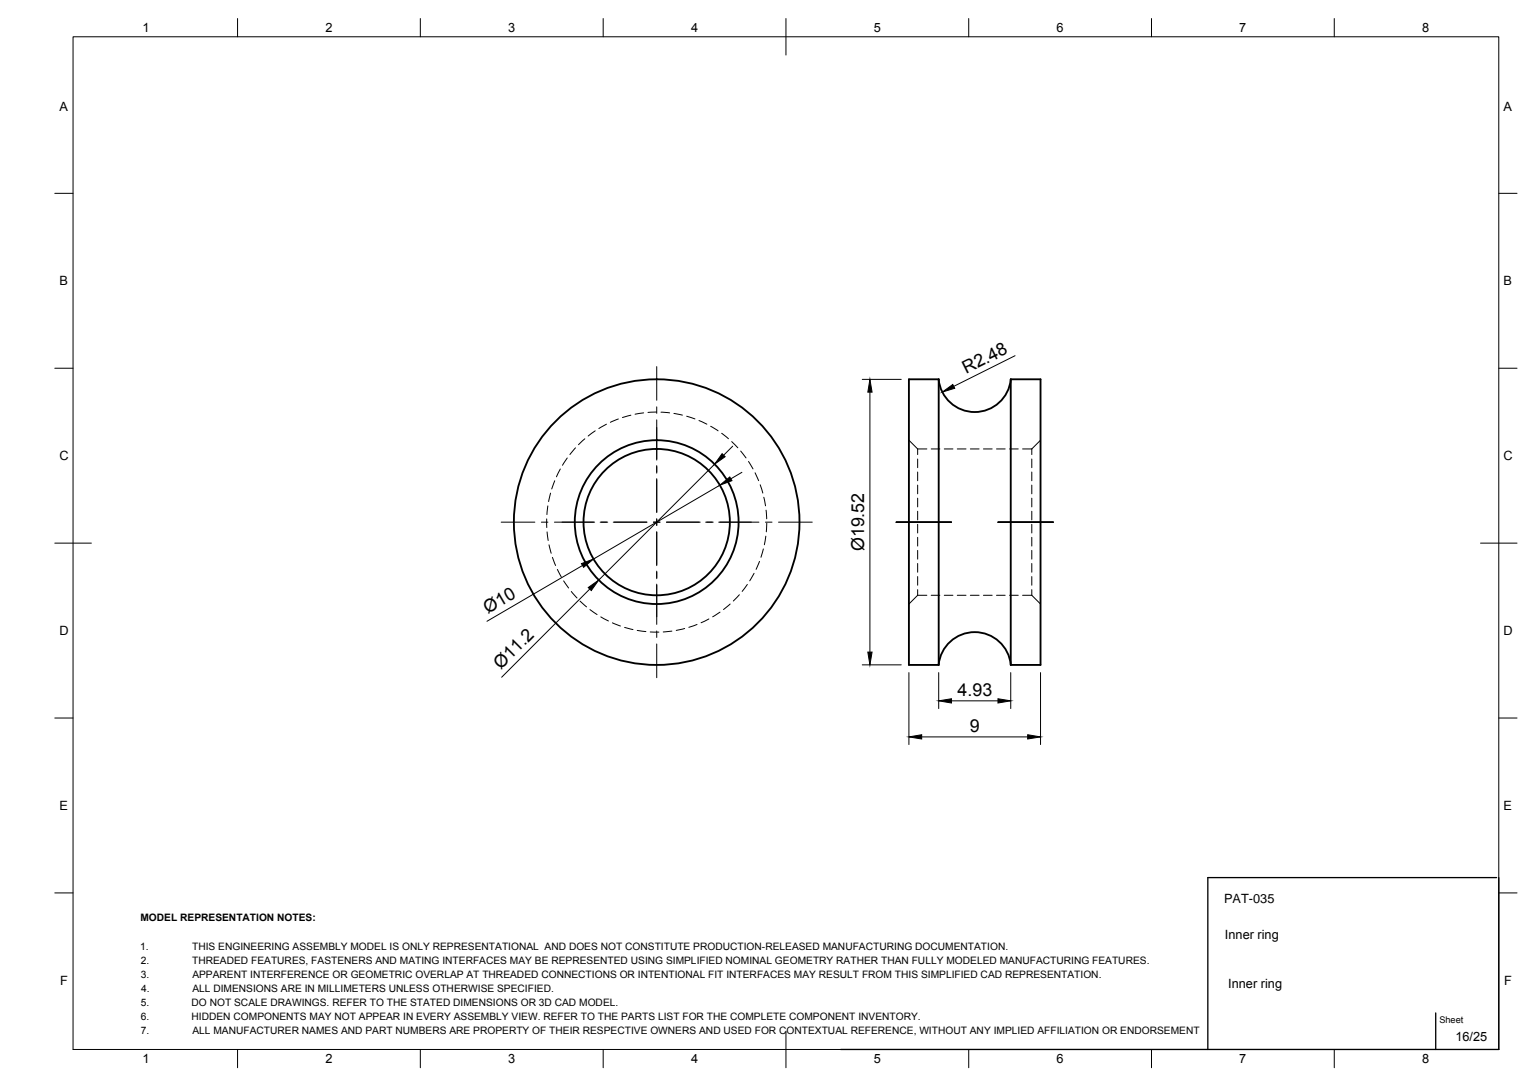
ISO-10303-21;
HEADER;
/* Generated by software containing ST-Developer
 * from STEP Tools, Inc. (www.steptools.com) 
 */

FILE_DESCRIPTION(
/* description */ ('Five-roller gravity conveyor'),
/* implementation_level */ '2;1');

FILE_NAME(
/* name */ 'Inner ring.step',
/* time_stamp */ '2026-10-29T15:36:43-07:00',
/* author */ (''),
/* organization */ (''),
/* preprocessor_version */ 'ST-DEVELOPER v20.2',
/* originating_system */ 'Autodesk Translation Framework v15.17.0.0',
/* authorisation */ '');

FILE_SCHEMA (('AUTOMOTIVE_DESIGN { 1 0 10303 214 3 1 1 }'));
ENDSEC;

DATA;
#10=MECHANICAL_DESIGN_GEOMETRIC_PRESENTATION_REPRESENTATION('',(#318),#7806);
#257=TOROIDAL_SURFACE('',#4620,1.,0.247676);
#264=CONICAL_SURFACE('',#4631,0.53,0.785398163397448);
#265=CONICAL_SURFACE('',#4638,0.53,0.785398163397448);
#282=SHAPE_REPRESENTATION_RELATIONSHIP('SRR','None',#7920,#300);
#300=ADVANCED_BREP_SHAPE_REPRESENTATION('',(#343),#7793);
#318=STYLED_ITEM('',(#8091),#343);
#343=MANIFOLD_SOLID_BREP('Body1',#4206);
#382=FACE_BOUND('',#1039,.T.);
#383=FACE_BOUND('',#1042,.T.);
#472=CIRCLE('',#4621,0.976185);
#473=CIRCLE('',#4622,0.976185);
#474=CIRCLE('',#4623,0.247676);
#475=CIRCLE('',#4624,0.976185);
#476=CIRCLE('',#4625,0.976185);
#477=CIRCLE('',#4627,0.976185);
#478=CIRCLE('',#4629,0.5);
#479=CIRCLE('',#4630,0.5);
#480=CIRCLE('',#4632,0.56);
#481=CIRCLE('',#4635,0.976185);
#482=CIRCLE('',#4637,0.56);
#617=CYLINDRICAL_SURFACE('',#4626,0.976185);
#618=CYLINDRICAL_SURFACE('',#4628,0.5);
#619=CYLINDRICAL_SURFACE('',#4634,0.976185);
#782=FACE_OUTER_BOUND('',#1034,.T.);
#783=FACE_OUTER_BOUND('',#1035,.T.);
#784=FACE_OUTER_BOUND('',#1036,.T.);
#785=FACE_OUTER_BOUND('',#1037,.T.);
#786=FACE_OUTER_BOUND('',#1038,.T.);
#787=FACE_OUTER_BOUND('',#1040,.T.);
#788=FACE_OUTER_BOUND('',#1041,.T.);
#789=FACE_OUTER_BOUND('',#1043,.T.);
#1034=EDGE_LOOP('',(#3420,#3421,#3422,#3423,#3424,#3425));
#1035=EDGE_LOOP('',(#3426,#3427,#3428,#3429,#3430));
#1036=EDGE_LOOP('',(#3431,#3432,#3433,#3434));
#1037=EDGE_LOOP('',(#3435,#3436,#3437,#3438));
#1038=EDGE_LOOP('',(#3439));
#1039=EDGE_LOOP('',(#3440));
#1040=EDGE_LOOP('',(#3441,#3442,#3443,#3444,#3445));
#1041=EDGE_LOOP('',(#3446));
#1042=EDGE_LOOP('',(#3447));
#1043=EDGE_LOOP('',(#3448,#3449,#3450,#3451));
#1455=LINE('',#6923,#1796);
#1456=LINE('',#6929,#1797);
#1457=LINE('',#6933,#1798);
#1458=LINE('',#6939,#1799);
#1459=LINE('',#6944,#1800);
#1796=VECTOR('',#5591,0.976185);
#1797=VECTOR('',#5598,0.5);
#1798=VECTOR('',#5603,0.53);
#1799=VECTOR('',#5612,0.976185);
#1800=VECTOR('',#5619,0.53);
#2078=VERTEX_POINT('',#6912);
#2079=VERTEX_POINT('',#6913);
#2080=VERTEX_POINT('',#6916);
#2081=VERTEX_POINT('',#6918);
#2082=VERTEX_POINT('',#6922);
#2083=VERTEX_POINT('',#6926);
#2084=VERTEX_POINT('',#6928);
#2085=VERTEX_POINT('',#6932);
#2086=VERTEX_POINT('',#6937);
#2087=VERTEX_POINT('',#6941);
#2553=EDGE_CURVE('',#2078,#2079,#472,.T.);
#2554=EDGE_CURVE('',#2079,#2078,#473,.T.);
#2555=EDGE_CURVE('',#2079,#2080,#474,.T.);
#2556=EDGE_CURVE('',#2081,#2080,#475,.T.);
#2557=EDGE_CURVE('',#2080,#2081,#476,.T.);
#2558=EDGE_CURVE('',#2081,#2082,#1455,.T.);
#2559=EDGE_CURVE('',#2082,#2082,#477,.T.);
#2560=EDGE_CURVE('',#2083,#2083,#478,.T.);
#2561=EDGE_CURVE('',#2083,#2084,#1456,.T.);
#2562=EDGE_CURVE('',#2084,#2084,#479,.T.);
#2563=EDGE_CURVE('',#2084,#2085,#1457,.T.);
#2564=EDGE_CURVE('',#2085,#2085,#480,.T.);
#2565=EDGE_CURVE('',#2086,#2086,#481,.T.);
#2566=EDGE_CURVE('',#2086,#2078,#1458,.T.);
#2567=EDGE_CURVE('',#2087,#2087,#482,.T.);
#2568=EDGE_CURVE('',#2087,#2083,#1459,.T.);
#3420=ORIENTED_EDGE('',*,*,#2553,.F.);
#3421=ORIENTED_EDGE('',*,*,#2554,.F.);
#3422=ORIENTED_EDGE('',*,*,#2555,.T.);
#3423=ORIENTED_EDGE('',*,*,#2556,.F.);
#3424=ORIENTED_EDGE('',*,*,#2557,.F.);
#3425=ORIENTED_EDGE('',*,*,#2555,.F.);
#3426=ORIENTED_EDGE('',*,*,#2556,.T.);
#3427=ORIENTED_EDGE('',*,*,#2557,.T.);
#3428=ORIENTED_EDGE('',*,*,#2558,.T.);
#3429=ORIENTED_EDGE('',*,*,#2559,.T.);
#3430=ORIENTED_EDGE('',*,*,#2558,.F.);
#3431=ORIENTED_EDGE('',*,*,#2560,.T.);
#3432=ORIENTED_EDGE('',*,*,#2561,.T.);
#3433=ORIENTED_EDGE('',*,*,#2562,.F.);
#3434=ORIENTED_EDGE('',*,*,#2561,.F.);
#3435=ORIENTED_EDGE('',*,*,#2562,.T.);
#3436=ORIENTED_EDGE('',*,*,#2563,.T.);
#3437=ORIENTED_EDGE('',*,*,#2564,.F.);
#3438=ORIENTED_EDGE('',*,*,#2563,.F.);
#3439=ORIENTED_EDGE('',*,*,#2559,.F.);
#3440=ORIENTED_EDGE('',*,*,#2564,.T.);
#3441=ORIENTED_EDGE('',*,*,#2565,.F.);
#3442=ORIENTED_EDGE('',*,*,#2566,.T.);
#3443=ORIENTED_EDGE('',*,*,#2553,.T.);
#3444=ORIENTED_EDGE('',*,*,#2554,.T.);
#3445=ORIENTED_EDGE('',*,*,#2566,.F.);
#3446=ORIENTED_EDGE('',*,*,#2565,.T.);
#3447=ORIENTED_EDGE('',*,*,#2567,.F.);
#3448=ORIENTED_EDGE('',*,*,#2567,.T.);
#3449=ORIENTED_EDGE('',*,*,#2568,.T.);
#3450=ORIENTED_EDGE('',*,*,#2560,.F.);
#3451=ORIENTED_EDGE('',*,*,#2568,.F.);
#3926=PLANE('',#4633);
#3927=PLANE('',#4636);
#4097=ADVANCED_FACE('',(#782),#257,.F.);
#4098=ADVANCED_FACE('',(#783),#617,.T.);
#4099=ADVANCED_FACE('',(#784),#618,.F.);
#4100=ADVANCED_FACE('',(#785),#264,.F.);
#4101=ADVANCED_FACE('',(#786,#382),#3926,.T.);
#4102=ADVANCED_FACE('',(#787),#619,.T.);
#4103=ADVANCED_FACE('',(#788,#383),#3927,.T.);
#4104=ADVANCED_FACE('',(#789),#265,.F.);
#4206=CLOSED_SHELL('',(#4097,#4098,#4099,#4100,#4101,#4102,#4103,#4104));
#4619=AXIS2_PLACEMENT_3D('',#6910,#5575,#5576);
#4620=AXIS2_PLACEMENT_3D('',#6911,#5577,#5578);
#4621=AXIS2_PLACEMENT_3D('',#6914,#5579,#5580);
#4622=AXIS2_PLACEMENT_3D('',#6915,#5581,#5582);
#4623=AXIS2_PLACEMENT_3D('',#6917,#5583,#5584);
#4624=AXIS2_PLACEMENT_3D('',#6919,#5585,#5586);
#4625=AXIS2_PLACEMENT_3D('',#6920,#5587,#5588);
#4626=AXIS2_PLACEMENT_3D('',#6921,#5589,#5590);
#4627=AXIS2_PLACEMENT_3D('',#6924,#5592,#5593);
#4628=AXIS2_PLACEMENT_3D('',#6925,#5594,#5595);
#4629=AXIS2_PLACEMENT_3D('',#6927,#5596,#5597);
#4630=AXIS2_PLACEMENT_3D('',#6930,#5599,#5600);
#4631=AXIS2_PLACEMENT_3D('',#6931,#5601,#5602);
#4632=AXIS2_PLACEMENT_3D('',#6934,#5604,#5605);
#4633=AXIS2_PLACEMENT_3D('',#6935,#5606,#5607);
#4634=AXIS2_PLACEMENT_3D('',#6936,#5608,#5609);
#4635=AXIS2_PLACEMENT_3D('',#6938,#5610,#5611);
#4636=AXIS2_PLACEMENT_3D('',#6940,#5613,#5614);
#4637=AXIS2_PLACEMENT_3D('',#6942,#5615,#5616);
#4638=AXIS2_PLACEMENT_3D('',#6943,#5617,#5618);
#5575=DIRECTION('axis',(0.,0.,1.));
#5576=DIRECTION('refdir',(1.,0.,0.));
#5577=DIRECTION('center_axis',(0.,-1.,0.));
#5578=DIRECTION('ref_axis',(0.,0.,-1.));
#5579=DIRECTION('center_axis',(0.,-1.,0.));
#5580=DIRECTION('ref_axis',(1.,0.,0.));
#5581=DIRECTION('center_axis',(0.,-1.,0.));
#5582=DIRECTION('ref_axis',(1.,0.,0.));
#5583=DIRECTION('center_axis',(1.,0.,1.22464679914735E-16));
#5584=DIRECTION('ref_axis',(-1.22464679914735E-16,0.,1.));
#5585=DIRECTION('center_axis',(0.,1.,0.));
#5586=DIRECTION('ref_axis',(1.,0.,0.));
#5587=DIRECTION('center_axis',(0.,1.,0.));
#5588=DIRECTION('ref_axis',(1.,0.,0.));
#5589=DIRECTION('center_axis',(0.,-1.,0.));
#5590=DIRECTION('ref_axis',(1.,0.,0.));
#5591=DIRECTION('',(0.,1.,0.));
#5592=DIRECTION('center_axis',(0.,-1.,0.));
#5593=DIRECTION('ref_axis',(1.,0.,0.));
#5594=DIRECTION('center_axis',(0.,-1.,0.));
#5595=DIRECTION('ref_axis',(1.,0.,0.));
#5596=DIRECTION('center_axis',(0.,-1.,0.));
#5597=DIRECTION('ref_axis',(1.,0.,0.));
#5598=DIRECTION('',(0.,1.,0.));
#5599=DIRECTION('center_axis',(0.,-1.,0.));
#5600=DIRECTION('ref_axis',(1.,0.,0.));
#5601=DIRECTION('center_axis',(0.,1.,0.));
#5602=DIRECTION('ref_axis',(1.,0.,0.));
#5603=DIRECTION('',(-0.707106781186547,0.707106781186548,-8.65956056235493E-17));
#5604=DIRECTION('center_axis',(0.,-1.,0.));
#5605=DIRECTION('ref_axis',(1.,0.,0.));
#5606=DIRECTION('center_axis',(0.,1.,0.));
#5607=DIRECTION('ref_axis',(0.,0.,1.));
#5608=DIRECTION('center_axis',(0.,-1.,0.));
#5609=DIRECTION('ref_axis',(1.,0.,0.));
#5610=DIRECTION('center_axis',(0.,-1.,0.));
#5611=DIRECTION('ref_axis',(1.,0.,0.));
#5612=DIRECTION('',(0.,1.,0.));
#5613=DIRECTION('center_axis',(0.,-1.,0.));
#5614=DIRECTION('ref_axis',(0.,0.,-1.));
#5615=DIRECTION('center_axis',(0.,-1.,0.));
#5616=DIRECTION('ref_axis',(1.,0.,0.));
#5617=DIRECTION('center_axis',(0.,-1.,0.));
#5618=DIRECTION('ref_axis',(1.,0.,0.));
#5619=DIRECTION('',(0.707106781186547,0.707106781186548,8.65956056235493E-17));
#6910=CARTESIAN_POINT('',(0.,0.,0.));
#6911=CARTESIAN_POINT('Origin',(0.,0.,0.));
#6912=CARTESIAN_POINT('',(-0.976185,-0.246528389340863,-1.19548183562566E-16));
#6913=CARTESIAN_POINT('',(-1.19548183562566E-16,-0.246528389340863,0.976185));
#6914=CARTESIAN_POINT('Origin',(0.,-0.246528389340863,0.));
#6915=CARTESIAN_POINT('Origin',(0.,-0.246528389340863,0.));
#6916=CARTESIAN_POINT('',(-1.19548183562566E-16,0.246528389340863,0.976185));
#6917=CARTESIAN_POINT('Origin',(-1.22464679914735E-16,0.,1.));
#6918=CARTESIAN_POINT('',(-0.976185,0.246528389340863,1.19548183562566E-16));
#6919=CARTESIAN_POINT('Origin',(0.,0.246528389340863,0.));
#6920=CARTESIAN_POINT('Origin',(0.,0.246528389340863,0.));
#6921=CARTESIAN_POINT('Origin',(0.,0.,0.));
#6922=CARTESIAN_POINT('',(-0.976185,0.45,-1.19548183562566E-16));
#6923=CARTESIAN_POINT('',(-0.976185,0.,-1.19548183562566E-16));
#6924=CARTESIAN_POINT('Origin',(0.,0.45,0.));
#6925=CARTESIAN_POINT('Origin',(0.,0.,0.));
#6926=CARTESIAN_POINT('',(-0.5,-0.39,-6.12323399573677E-17));
#6927=CARTESIAN_POINT('Origin',(0.,-0.39,0.));
#6928=CARTESIAN_POINT('',(-0.5,0.39,-6.12323399573677E-17));
#6929=CARTESIAN_POINT('',(-0.5,0.,-6.12323399573677E-17));
#6930=CARTESIAN_POINT('Origin',(0.,0.39,0.));
#6931=CARTESIAN_POINT('Origin',(0.,0.42,0.));
#6932=CARTESIAN_POINT('',(-0.56,0.45,-6.85802207522518E-17));
#6933=CARTESIAN_POINT('',(-0.53,0.42,-6.49062803548097E-17));
#6934=CARTESIAN_POINT('Origin',(0.,0.45,0.));
#6935=CARTESIAN_POINT('Origin',(0.976185,0.45,0.));
#6936=CARTESIAN_POINT('Origin',(0.,0.,0.));
#6937=CARTESIAN_POINT('',(-0.976185,-0.45,-1.19548183562566E-16));
#6938=CARTESIAN_POINT('Origin',(0.,-0.45,0.));
#6939=CARTESIAN_POINT('',(-0.976185,0.,-1.19548183562566E-16));
#6940=CARTESIAN_POINT('Origin',(0.56,-0.45,0.));
#6941=CARTESIAN_POINT('',(-0.56,-0.45,-6.85802207522518E-17));
#6942=CARTESIAN_POINT('Origin',(0.,-0.45,0.));
#6943=CARTESIAN_POINT('Origin',(0.,-0.42,0.));
#6944=CARTESIAN_POINT('',(-0.53,-0.42,-6.49062803548097E-17));
#7769=UNCERTAINTY_MEASURE_WITH_UNIT(LENGTH_MEASURE(0.001),#7807,
'DISTANCE_ACCURACY_VALUE',
'Maximum model space distance between geometric entities at asserted c
onnectivities');
#7782=UNCERTAINTY_MEASURE_WITH_UNIT(LENGTH_MEASURE(0.001),#7807,
'DISTANCE_ACCURACY_VALUE',
'Maximum model space distance between geometric entities at asserted c
onnectivities');
#7793=(
GEOMETRIC_REPRESENTATION_CONTEXT(3)
GLOBAL_UNCERTAINTY_ASSIGNED_CONTEXT((#7769))
GLOBAL_UNIT_ASSIGNED_CONTEXT((#7807,#7809,#7810))
REPRESENTATION_CONTEXT('','3D')
);
#7806=(
GEOMETRIC_REPRESENTATION_CONTEXT(3)
GLOBAL_UNCERTAINTY_ASSIGNED_CONTEXT((#7782))
GLOBAL_UNIT_ASSIGNED_CONTEXT((#7807,#7809,#7810))
REPRESENTATION_CONTEXT('','3D')
);
#7807=(
LENGTH_UNIT()
NAMED_UNIT(*)
SI_UNIT(.CENTI.,.METRE.)
);
#7809=(
NAMED_UNIT(*)
PLANE_ANGLE_UNIT()
SI_UNIT($,.RADIAN.)
);
#7810=(
NAMED_UNIT(*)
SI_UNIT($,.STERADIAN.)
SOLID_ANGLE_UNIT()
);
#7821=SHAPE_DEFINITION_REPRESENTATION(#7844,#7920);
#7844=PRODUCT_DEFINITION_SHAPE('',$,#7944);
#7920=SHAPE_REPRESENTATION('',(#4619),#7793);
#7933=PRODUCT_DEFINITION_CONTEXT('part definition',#8004,'design');
#7944=PRODUCT_DEFINITION('Inner ring','Inner ring',#7967,#7933);
#7967=PRODUCT_DEFINITION_FORMATION('',$,#8016);
#8004=APPLICATION_CONTEXT(
'Core Data for Automotive Mechanical Design Process');
#8005=PRODUCT_CONTEXT('part definition',#8004,'mechanical');
#8016=PRODUCT('Inner ring','Inner ring','Inner ring',(#8005));
#8085=COLOUR_RGB('Grey',0.48,0.52,0.57);
#8086=FILL_AREA_STYLE_COLOUR('',#8085);
#8087=FILL_AREA_STYLE('',(#8086));
#8088=SURFACE_STYLE_FILL_AREA(#8087);
#8089=SURFACE_SIDE_STYLE('',(#8088));
#8090=SURFACE_STYLE_USAGE(.BOTH.,#8089);
#8091=PRESENTATION_STYLE_ASSIGNMENT((#8090));
ENDSEC;
END-ISO-10303-21;
